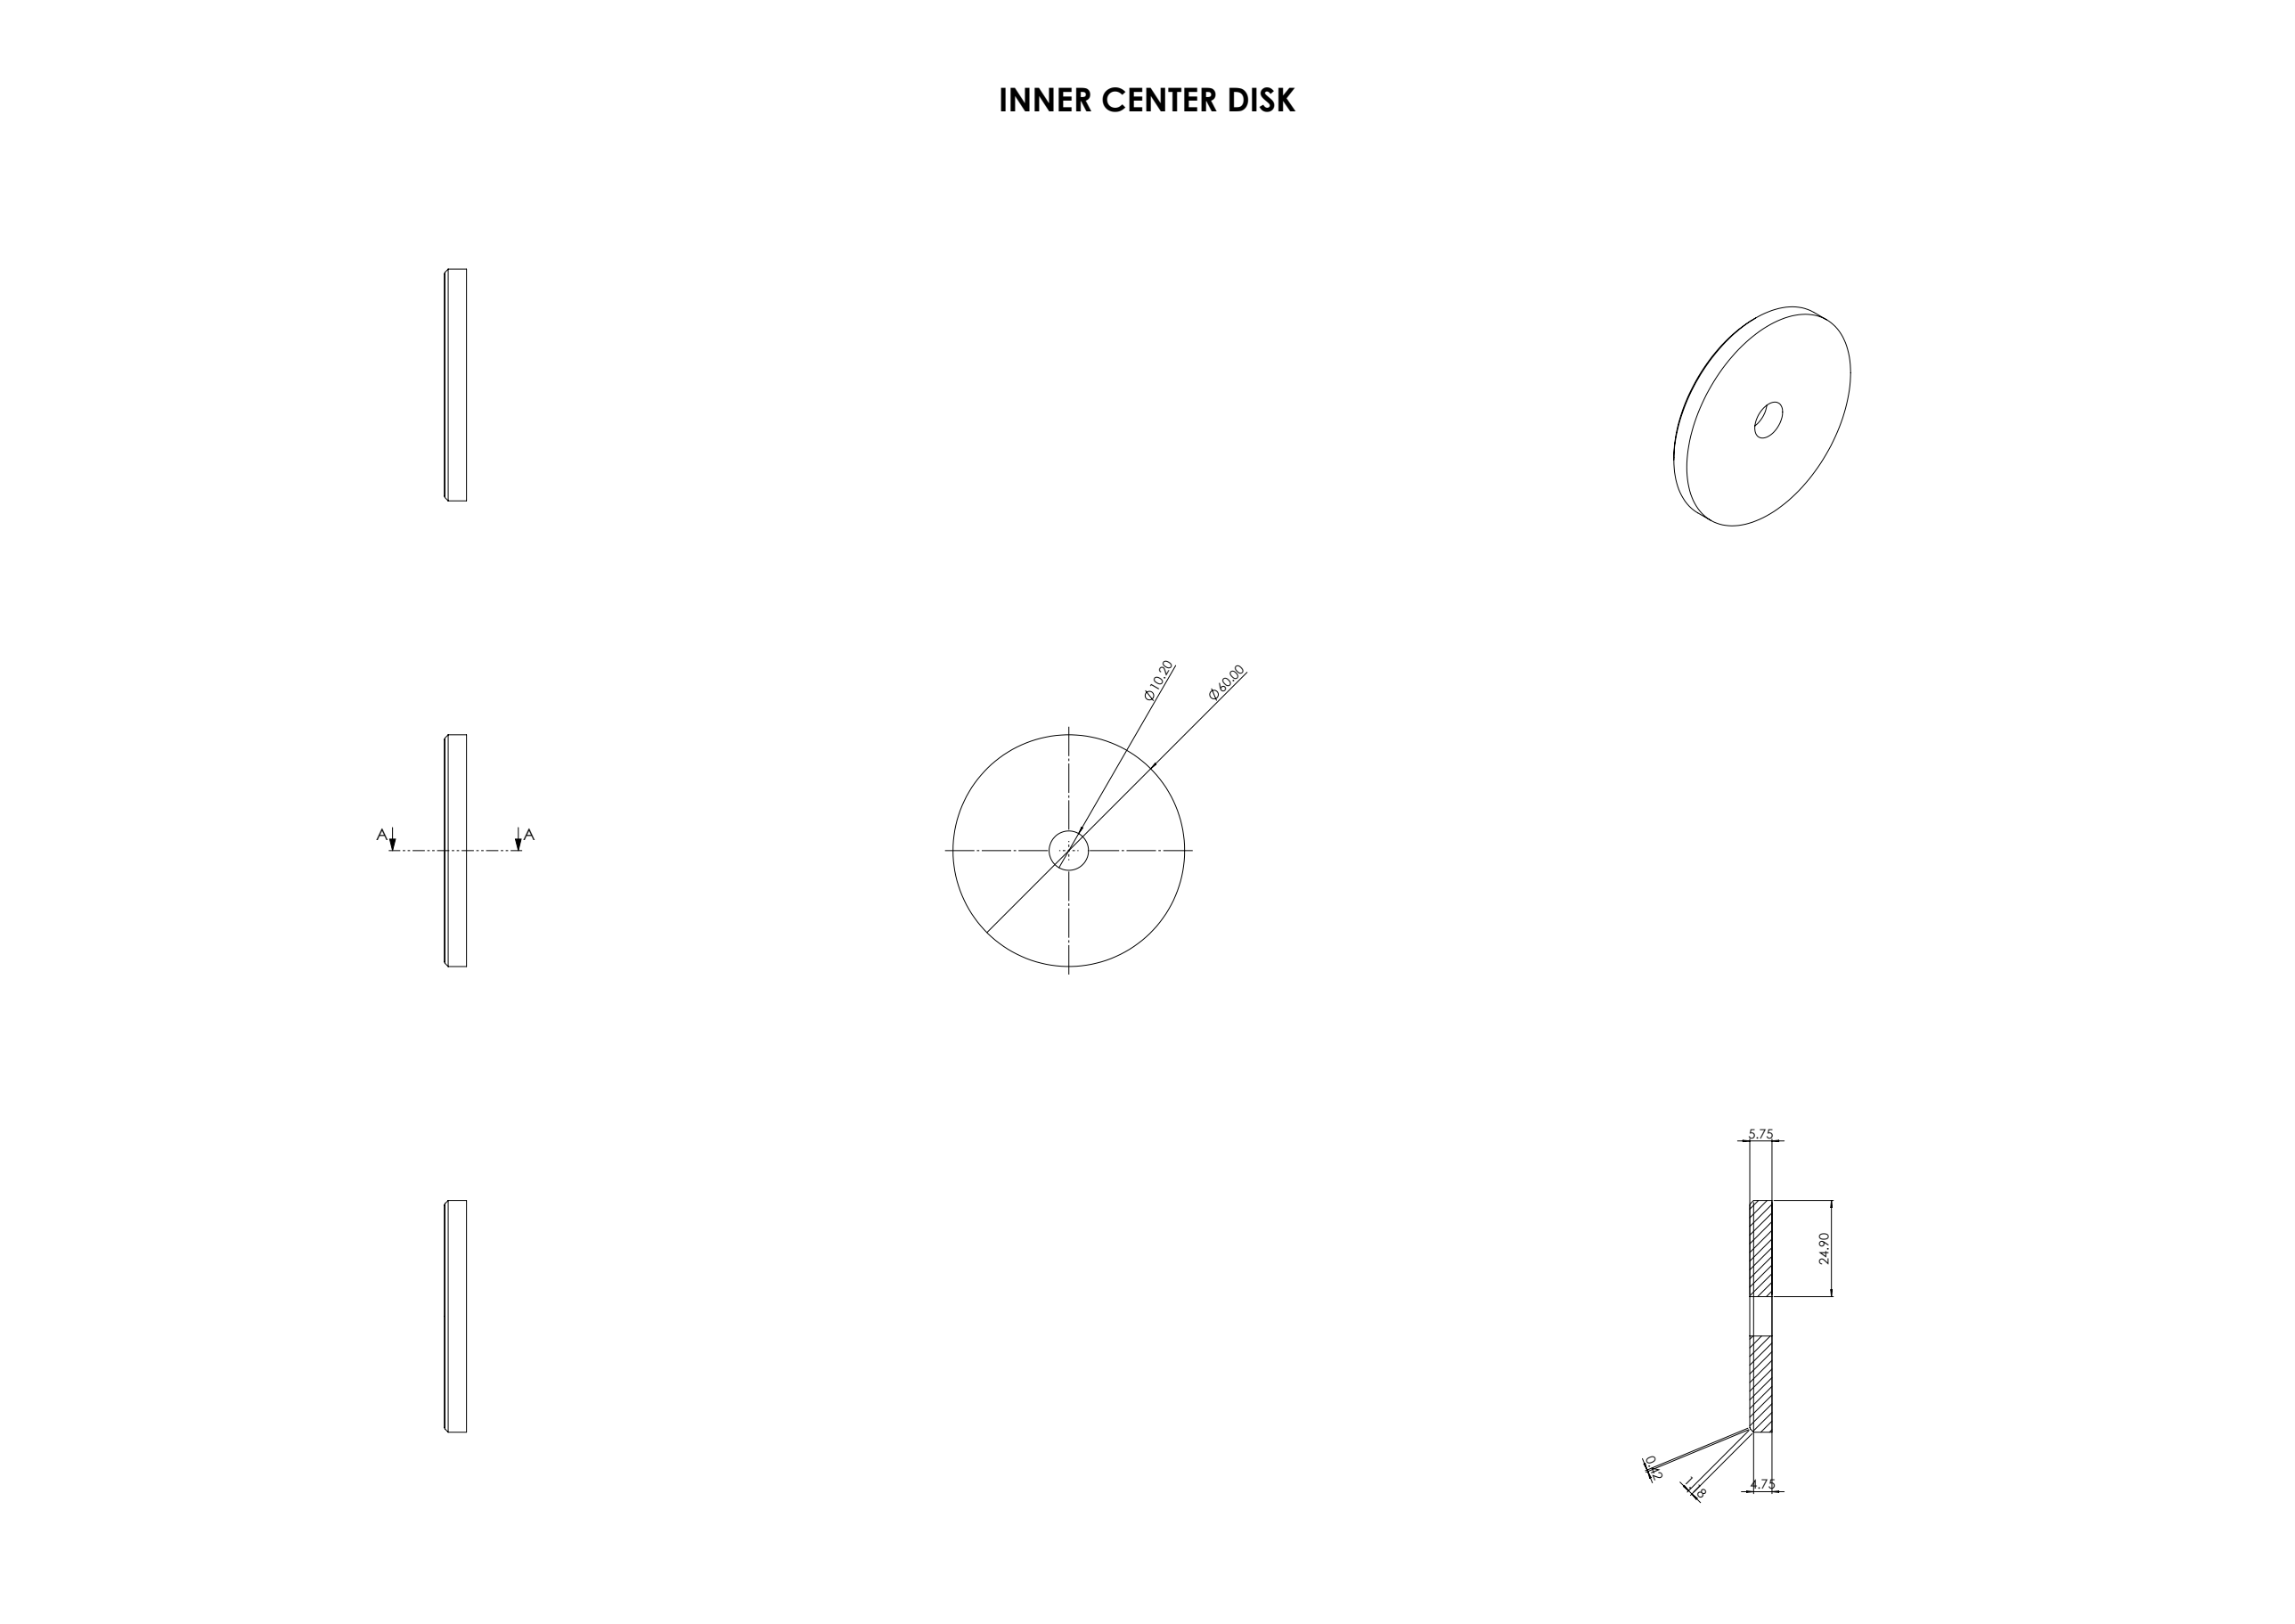
ISO-10303-21;
HEADER;
/* Generated by software containing ST-Developer
 * from STEP Tools, Inc. (www.steptools.com) 
 */

FILE_DESCRIPTION(
/* description */ (''),
/* implementation_level */ '2;1');

FILE_NAME(
/* name */ '06_Inner_Center_Disk.step',
/* time_stamp */ '2026-10-26T06:13:19-07:00',
/* author */ (''),
/* organization */ (''),
/* preprocessor_version */ 'ST-DEVELOPER v20.2',
/* originating_system */ 'Autodesk Translation Framework v15.15.0.0',
/* authorisation */ '');

FILE_SCHEMA (('AUTOMOTIVE_DESIGN { 1 0 10303 214 3 1 1 }','TECHNICAL_DATA_PACKAGING'));
ENDSEC;

DATA;
#10=MECHANICAL_DESIGN_GEOMETRIC_PRESENTATION_REPRESENTATION('',(#302),#56639);
#262=SHAPE_REPRESENTATION_RELATIONSHIP('SRR','None',#56750,#282);
#282=ADVANCED_BREP_SHAPE_REPRESENTATION('',(#322),#56624);
#302=STYLED_ITEM('',(#56929),#322);
#322=MANIFOLD_SOLID_BREP('Body1',#16954);
#506=FACE_BOUND('',#3082,.T.);
#507=FACE_BOUND('',#3087,.T.);
#589=CONICAL_SURFACE('',#17651,28.9663172798365,1.17809724509618);
#590=CONICAL_SURFACE('',#17657,29.5,0.785398163397448);
#908=CIRCLE('',#17652,29.1626345596729);
#909=CIRCLE('',#17653,29.1626345596729);
#910=CIRCLE('',#17654,28.77);
#911=CIRCLE('',#17656,5.1);
#912=CIRCLE('',#17658,30.);
#913=CIRCLE('',#17660,5.1);
#914=CIRCLE('',#17662,30.);
#1317=CYLINDRICAL_SURFACE('',#17659,5.1);
#1318=CYLINDRICAL_SURFACE('',#17661,30.);
#2015=FACE_OUTER_BOUND('',#3080,.T.);
#2016=FACE_OUTER_BOUND('',#3081,.T.);
#2017=FACE_OUTER_BOUND('',#3083,.T.);
#2018=FACE_OUTER_BOUND('',#3084,.T.);
#2019=FACE_OUTER_BOUND('',#3085,.T.);
#2020=FACE_OUTER_BOUND('',#3086,.T.);
#3080=EDGE_LOOP('',(#11792,#11793,#11794,#11795,#11796));
#3081=EDGE_LOOP('',(#11797));
#3082=EDGE_LOOP('',(#11798));
#3083=EDGE_LOOP('',(#11799,#11800,#11801,#11802,#11803));
#3084=EDGE_LOOP('',(#11804,#11805,#11806,#11807));
#3085=EDGE_LOOP('',(#11808,#11809,#11810,#11811));
#3086=EDGE_LOOP('',(#11812));
#3087=EDGE_LOOP('',(#11813));
#4093=LINE('',#25066,#5047);
#4094=LINE('',#25074,#5048);
#4095=LINE('',#25078,#5049);
#4096=LINE('',#25082,#5050);
#5047=VECTOR('',#19909,28.9663172798364);
#5048=VECTOR('',#19920,29.5);
#5049=VECTOR('',#19925,5.1);
#5050=VECTOR('',#19930,30.);
#7039=VERTEX_POINT('',#25061);
#7040=VERTEX_POINT('',#25062);
#7041=VERTEX_POINT('',#25065);
#7042=VERTEX_POINT('',#25069);
#7043=VERTEX_POINT('',#25072);
#7044=VERTEX_POINT('',#25076);
#7045=VERTEX_POINT('',#25080);
#8803=EDGE_CURVE('',#7039,#7040,#908,.T.);
#8804=EDGE_CURVE('',#7040,#7039,#909,.T.);
#8805=EDGE_CURVE('',#7039,#7041,#4093,.T.);
#8806=EDGE_CURVE('',#7041,#7041,#910,.T.);
#8807=EDGE_CURVE('',#7042,#7042,#911,.T.);
#8808=EDGE_CURVE('',#7043,#7043,#912,.T.);
#8809=EDGE_CURVE('',#7043,#7040,#4094,.T.);
#8810=EDGE_CURVE('',#7044,#7044,#913,.T.);
#8811=EDGE_CURVE('',#7044,#7042,#4095,.T.);
#8812=EDGE_CURVE('',#7045,#7045,#914,.T.);
#8813=EDGE_CURVE('',#7045,#7043,#4096,.T.);
#11792=ORIENTED_EDGE('',*,*,#8803,.T.);
#11793=ORIENTED_EDGE('',*,*,#8804,.T.);
#11794=ORIENTED_EDGE('',*,*,#8805,.T.);
#11795=ORIENTED_EDGE('',*,*,#8806,.T.);
#11796=ORIENTED_EDGE('',*,*,#8805,.F.);
#11797=ORIENTED_EDGE('',*,*,#8806,.F.);
#11798=ORIENTED_EDGE('',*,*,#8807,.T.);
#11799=ORIENTED_EDGE('',*,*,#8808,.F.);
#11800=ORIENTED_EDGE('',*,*,#8809,.T.);
#11801=ORIENTED_EDGE('',*,*,#8803,.F.);
#11802=ORIENTED_EDGE('',*,*,#8804,.F.);
#11803=ORIENTED_EDGE('',*,*,#8809,.F.);
#11804=ORIENTED_EDGE('',*,*,#8810,.T.);
#11805=ORIENTED_EDGE('',*,*,#8811,.T.);
#11806=ORIENTED_EDGE('',*,*,#8807,.F.);
#11807=ORIENTED_EDGE('',*,*,#8811,.F.);
#11808=ORIENTED_EDGE('',*,*,#8812,.F.);
#11809=ORIENTED_EDGE('',*,*,#8813,.T.);
#11810=ORIENTED_EDGE('',*,*,#8808,.T.);
#11811=ORIENTED_EDGE('',*,*,#8813,.F.);
#11812=ORIENTED_EDGE('',*,*,#8812,.T.);
#11813=ORIENTED_EDGE('',*,*,#8810,.F.);
#15779=PLANE('',#17655);
#15780=PLANE('',#17663);
#16186=ADVANCED_FACE('',(#2015),#589,.T.);
#16187=ADVANCED_FACE('',(#2016,#506),#15779,.T.);
#16188=ADVANCED_FACE('',(#2017),#590,.T.);
#16189=ADVANCED_FACE('',(#2018),#1317,.F.);
#16190=ADVANCED_FACE('',(#2019),#1318,.T.);
#16191=ADVANCED_FACE('',(#2020,#507),#15780,.T.);
#16954=CLOSED_SHELL('',(#16186,#16187,#16188,#16189,#16190,#16191));
#17650=AXIS2_PLACEMENT_3D('',#25059,#19901,#19902);
#17651=AXIS2_PLACEMENT_3D('',#25060,#19903,#19904);
#17652=AXIS2_PLACEMENT_3D('',#25063,#19905,#19906);
#17653=AXIS2_PLACEMENT_3D('',#25064,#19907,#19908);
#17654=AXIS2_PLACEMENT_3D('',#25067,#19910,#19911);
#17655=AXIS2_PLACEMENT_3D('',#25068,#19912,#19913);
#17656=AXIS2_PLACEMENT_3D('',#25070,#19914,#19915);
#17657=AXIS2_PLACEMENT_3D('',#25071,#19916,#19917);
#17658=AXIS2_PLACEMENT_3D('',#25073,#19918,#19919);
#17659=AXIS2_PLACEMENT_3D('',#25075,#19921,#19922);
#17660=AXIS2_PLACEMENT_3D('',#25077,#19923,#19924);
#17661=AXIS2_PLACEMENT_3D('',#25079,#19926,#19927);
#17662=AXIS2_PLACEMENT_3D('',#25081,#19928,#19929);
#17663=AXIS2_PLACEMENT_3D('',#25083,#19931,#19932);
#19901=DIRECTION('axis',(0.,0.,1.));
#19902=DIRECTION('refdir',(1.,0.,0.));
#19903=DIRECTION('center_axis',(1.,0.,-1.09798087011876E-14));
#19904=DIRECTION('ref_axis',(0.,-1.,-3.08236690249437E-17));
#19905=DIRECTION('center_axis',(-1.,0.,0.));
#19906=DIRECTION('ref_axis',(0.,-1.,-6.12323399573677E-17));
#19907=DIRECTION('center_axis',(-1.,0.,0.));
#19908=DIRECTION('ref_axis',(0.,-1.,-6.12323399573677E-17));
#19909=DIRECTION('',(-0.382683432365084,-0.923879532511289,4.06017091232465E-15));
#19910=DIRECTION('center_axis',(1.,0.,0.));
#19911=DIRECTION('ref_axis',(0.,-1.,0.));
#19912=DIRECTION('center_axis',(-1.,0.,0.));
#19913=DIRECTION('ref_axis',(0.,0.,1.));
#19914=DIRECTION('center_axis',(1.,0.,0.));
#19915=DIRECTION('ref_axis',(0.,0.,-1.));
#19916=DIRECTION('center_axis',(1.,0.,0.));
#19917=DIRECTION('ref_axis',(0.,1.,0.));
#19918=DIRECTION('center_axis',(1.,0.,0.));
#19919=DIRECTION('ref_axis',(0.,0.,-1.));
#19920=DIRECTION('',(-0.707106781186547,0.707106781186548,8.65956056235493E-17));
#19921=DIRECTION('center_axis',(1.,0.,0.));
#19922=DIRECTION('ref_axis',(0.,1.,0.));
#19923=DIRECTION('center_axis',(1.,0.,0.));
#19924=DIRECTION('ref_axis',(0.,0.,-1.));
#19925=DIRECTION('',(-1.,0.,0.));
#19926=DIRECTION('center_axis',(1.,0.,0.));
#19927=DIRECTION('ref_axis',(0.,1.,0.));
#19928=DIRECTION('center_axis',(1.,0.,0.));
#19929=DIRECTION('ref_axis',(0.,0.,-1.));
#19930=DIRECTION('',(-1.,0.,0.));
#19931=DIRECTION('center_axis',(1.,0.,0.));
#19932=DIRECTION('ref_axis',(0.,0.,-1.));
#25059=CARTESIAN_POINT('',(0.,0.,0.));
#25060=CARTESIAN_POINT('Origin',(30.0813172798365,0.,-8.92848176705185E-16));
#25061=CARTESIAN_POINT('',(30.1626345596729,29.1626345596729,-3.57139270682074E-15));
#25062=CARTESIAN_POINT('',(30.1626345596729,-29.1626345596729,-3.57139270682074E-15));
#25063=CARTESIAN_POINT('Origin',(30.1626345596729,0.,-1.78569635341037E-15));
#25064=CARTESIAN_POINT('Origin',(30.1626345596729,0.,-1.78569635341037E-15));
#25065=CARTESIAN_POINT('',(30.,28.77,3.52330884114693E-15));
#25066=CARTESIAN_POINT('',(30.0813172798365,28.9663172798365,3.54735077398384E-15));
#25067=CARTESIAN_POINT('Origin',(30.,0.,0.));
#25068=CARTESIAN_POINT('Origin',(30.,29.,0.));
#25069=CARTESIAN_POINT('',(30.,-5.1,-6.2456986756515E-16));
#25070=CARTESIAN_POINT('Origin',(30.,0.,0.));
#25071=CARTESIAN_POINT('Origin',(30.5,0.,0.));
#25072=CARTESIAN_POINT('',(31.,-30.,-3.67394039744206E-15));
#25073=CARTESIAN_POINT('Origin',(31.,0.,0.));
#25074=CARTESIAN_POINT('',(30.5,-29.5,-3.61270805748469E-15));
#25075=CARTESIAN_POINT('Origin',(32.875,0.,0.));
#25076=CARTESIAN_POINT('',(35.75,-5.1,-6.2456986756515E-16));
#25077=CARTESIAN_POINT('Origin',(35.75,0.,0.));
#25078=CARTESIAN_POINT('',(32.875,-5.1,-6.2456986756515E-16));
#25079=CARTESIAN_POINT('Origin',(33.375,0.,0.));
#25080=CARTESIAN_POINT('',(35.75,-30.,-3.67394039744206E-15));
#25081=CARTESIAN_POINT('Origin',(35.75,0.,0.));
#25082=CARTESIAN_POINT('',(33.375,-30.,-3.67394039744206E-15));
#25083=CARTESIAN_POINT('Origin',(35.75,5.1,0.));
#56602=UNCERTAINTY_MEASURE_WITH_UNIT(LENGTH_MEASURE(0.01),#56640,
'DISTANCE_ACCURACY_VALUE',
'Maximum model space distance between geometric entities at asserted c
onnectivities');
#56617=UNCERTAINTY_MEASURE_WITH_UNIT(LENGTH_MEASURE(0.01),#56640,
'DISTANCE_ACCURACY_VALUE',
'Maximum model space distance between geometric entities at asserted c
onnectivities');
#56624=(
GEOMETRIC_REPRESENTATION_CONTEXT(3)
GLOBAL_UNCERTAINTY_ASSIGNED_CONTEXT((#56602))
GLOBAL_UNIT_ASSIGNED_CONTEXT((#56640,#56642,#56643))
REPRESENTATION_CONTEXT('','3D')
);
#56639=(
GEOMETRIC_REPRESENTATION_CONTEXT(3)
GLOBAL_UNCERTAINTY_ASSIGNED_CONTEXT((#56617))
GLOBAL_UNIT_ASSIGNED_CONTEXT((#56640,#56642,#56643))
REPRESENTATION_CONTEXT('','3D')
);
#56640=(
LENGTH_UNIT()
NAMED_UNIT(*)
SI_UNIT(.MILLI.,.METRE.)
);
#56642=(
NAMED_UNIT(*)
PLANE_ANGLE_UNIT()
SI_UNIT($,.RADIAN.)
);
#56643=(
NAMED_UNIT(*)
SI_UNIT($,.STERADIAN.)
SOLID_ANGLE_UNIT()
);
#56650=SHAPE_DEFINITION_REPRESENTATION(#56671,#56750);
#56671=PRODUCT_DEFINITION_SHAPE('',$,#56772);
#56750=SHAPE_REPRESENTATION('',(#17650),#56624);
#56765=PRODUCT_DEFINITION_CONTEXT('part definition',#56830,'design');
#56772=PRODUCT_DEFINITION('2026-10-26-00-02-42-220',
'06_Inner_Center_Disk',#56793,#56765);
#56793=PRODUCT_DEFINITION_FORMATION('',$,#56838);
#56830=APPLICATION_CONTEXT(
'Core Data for Automotive Mechanical Design Process');
#56831=PRODUCT_CONTEXT('part definition',#56830,'mechanical');
#56838=PRODUCT('2026-10-26-00-02-42-220','06_Inner_Center_Disk',$,(#56831));
#56923=COLOUR_RGB('Off White',0.89,0.88,0.83);
#56924=FILL_AREA_STYLE_COLOUR('',#56923);
#56925=FILL_AREA_STYLE('',(#56924));
#56926=SURFACE_STYLE_FILL_AREA(#56925);
#56927=SURFACE_SIDE_STYLE('',(#56926));
#56928=SURFACE_STYLE_USAGE(.BOTH.,#56927);
#56929=PRESENTATION_STYLE_ASSIGNMENT((#56928));
ENDSEC;
END-ISO-10303-21;
